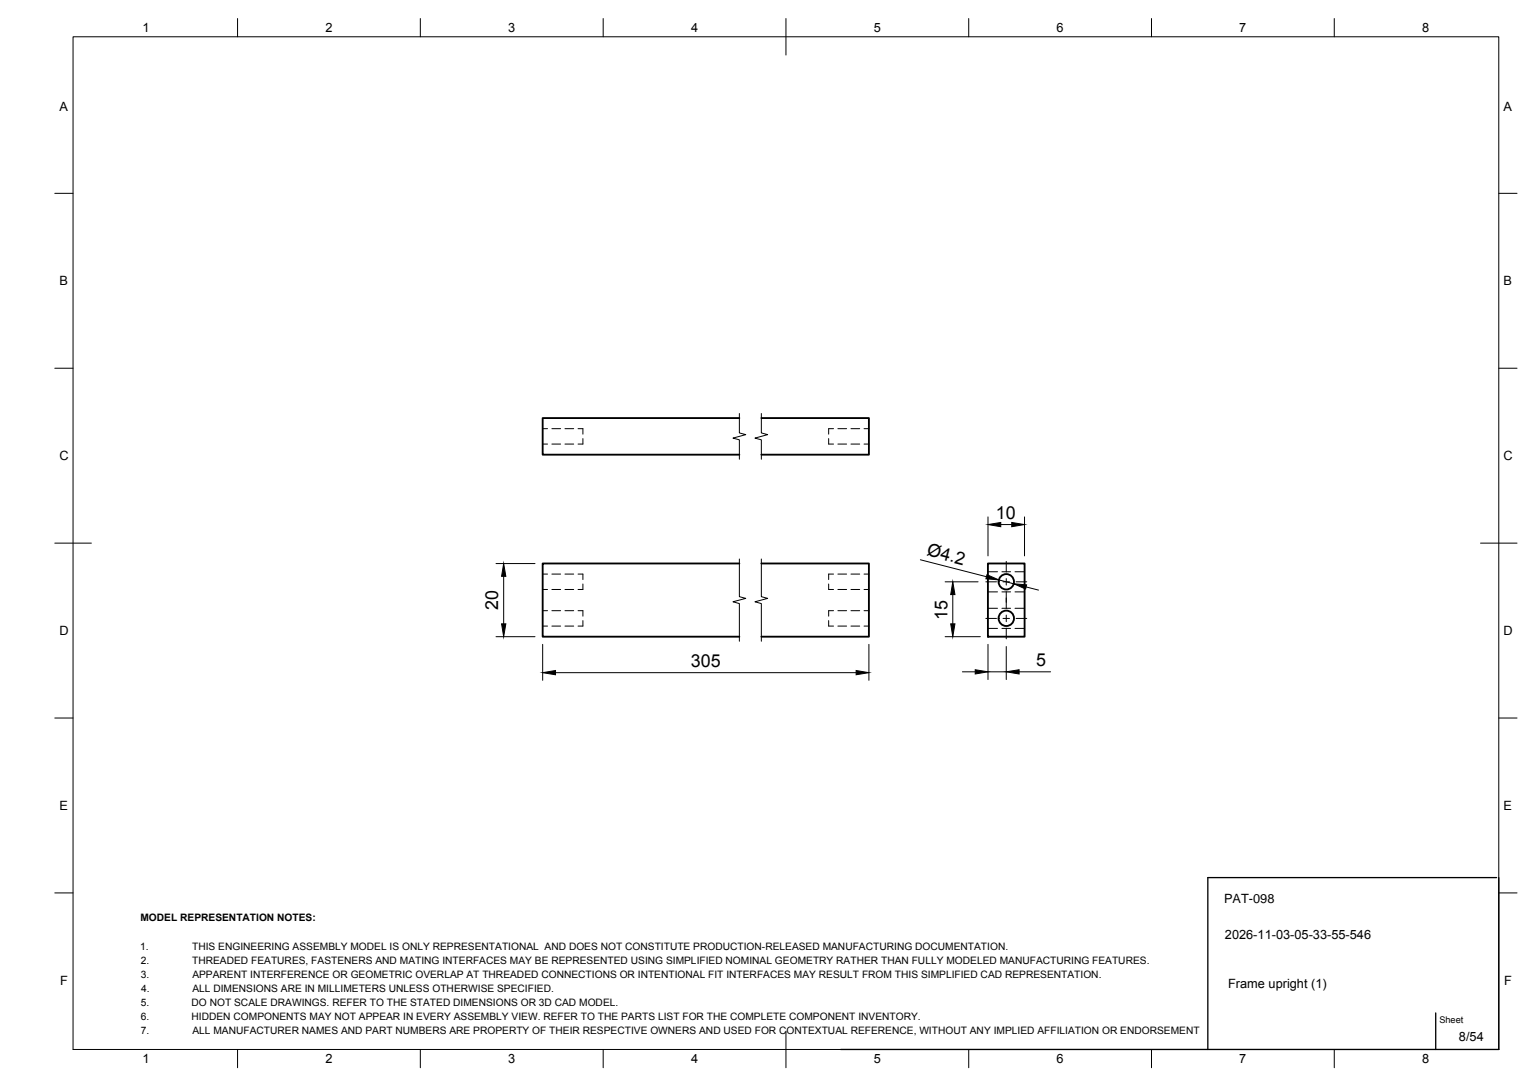
ISO-10303-21;
HEADER;
/* Generated by software containing ST-Developer
 * from STEP Tools, Inc. (www.steptools.com) 
 */

FILE_DESCRIPTION(
/* description */ ('Spring compression tester'),
/* implementation_level */ '2;1');

FILE_NAME(
/* name */ 'Frame upright (1).step',
/* time_stamp */ '2026-10-28T03:24:11-07:00',
/* author */ (''),
/* organization */ (''),
/* preprocessor_version */ 'ST-DEVELOPER v20.2',
/* originating_system */ 'Autodesk Translation Framework v15.17.0.0',
/* authorisation */ '');

FILE_SCHEMA (('AUTOMOTIVE_DESIGN { 1 0 10303 214 3 1 1 }'));
ENDSEC;

DATA;
#10=MECHANICAL_DESIGN_GEOMETRIC_PRESENTATION_REPRESENTATION('',(#1109),#43521);
#989=SHAPE_REPRESENTATION_RELATIONSHIP('SRR','None',#43801,#1049);
#1049=ADVANCED_BREP_SHAPE_REPRESENTATION('',(#1184),#43461);
#1109=STYLED_ITEM('',(#44181),#1184);
#1184=MANIFOLD_SOLID_BREP('Body1',#18546);
#1313=FACE_BOUND('',#3377,.T.);
#1314=FACE_BOUND('',#3378,.T.);
#1315=FACE_BOUND('',#3381,.T.);
#1316=FACE_BOUND('',#3382,.T.);
#1317=FACE_BOUND('',#3384,.T.);
#1318=FACE_BOUND('',#3385,.T.);
#1319=FACE_BOUND('',#3387,.T.);
#1320=FACE_BOUND('',#3388,.T.);
#1635=PLANE('',#19455);
#1636=PLANE('',#19459);
#1637=PLANE('',#19463);
#1638=PLANE('',#19467);
#1639=PLANE('',#19468);
#1640=PLANE('',#19469);
#1641=PLANE('',#19470);
#1642=PLANE('',#19471);
#1643=PLANE('',#19472);
#1644=PLANE('',#19473);
#2252=FACE_OUTER_BOUND('',#3365,.T.);
#2253=FACE_OUTER_BOUND('',#3366,.T.);
#2254=FACE_OUTER_BOUND('',#3367,.T.);
#2255=FACE_OUTER_BOUND('',#3368,.T.);
#2256=FACE_OUTER_BOUND('',#3369,.T.);
#2257=FACE_OUTER_BOUND('',#3370,.T.);
#2258=FACE_OUTER_BOUND('',#3371,.T.);
#2259=FACE_OUTER_BOUND('',#3372,.T.);
#2260=FACE_OUTER_BOUND('',#3373,.T.);
#2261=FACE_OUTER_BOUND('',#3374,.T.);
#2262=FACE_OUTER_BOUND('',#3375,.T.);
#2263=FACE_OUTER_BOUND('',#3376,.T.);
#2264=FACE_OUTER_BOUND('',#3379,.T.);
#2265=FACE_OUTER_BOUND('',#3380,.T.);
#2266=FACE_OUTER_BOUND('',#3383,.T.);
#2267=FACE_OUTER_BOUND('',#3386,.T.);
#3365=EDGE_LOOP('',(#12601,#12602,#12603,#12604));
#3366=EDGE_LOOP('',(#12605,#12606,#12607,#12608));
#3367=EDGE_LOOP('',(#12609,#12610,#12611,#12612));
#3368=EDGE_LOOP('',(#12613));
#3369=EDGE_LOOP('',(#12614,#12615,#12616,#12617));
#3370=EDGE_LOOP('',(#12618));
#3371=EDGE_LOOP('',(#12619,#12620,#12621,#12622));
#3372=EDGE_LOOP('',(#12623));
#3373=EDGE_LOOP('',(#12624,#12625,#12626,#12627));
#3374=EDGE_LOOP('',(#12628));
#3375=EDGE_LOOP('',(#12629,#12630,#12631,#12632));
#3376=EDGE_LOOP('',(#12633,#12634,#12635,#12636));
#3377=EDGE_LOOP('',(#12637));
#3378=EDGE_LOOP('',(#12638));
#3379=EDGE_LOOP('',(#12639,#12640,#12641,#12642));
#3380=EDGE_LOOP('',(#12643,#12644,#12645,#12646));
#3381=EDGE_LOOP('',(#12647));
#3382=EDGE_LOOP('',(#12648));
#3383=EDGE_LOOP('',(#12649,#12650,#12651,#12652));
#3384=EDGE_LOOP('',(#12653));
#3385=EDGE_LOOP('',(#12654));
#3386=EDGE_LOOP('',(#12655,#12656,#12657,#12658));
#3387=EDGE_LOOP('',(#12659));
#3388=EDGE_LOOP('',(#12660));
#4726=LINE('',#26866,#6158);
#4727=LINE('',#26872,#6159);
#4728=LINE('',#26878,#6160);
#4729=LINE('',#26885,#6161);
#4730=LINE('',#26892,#6162);
#4731=LINE('',#26899,#6163);
#4732=LINE('',#26905,#6164);
#4733=LINE('',#26907,#6165);
#4734=LINE('',#26909,#6166);
#4735=LINE('',#26910,#6167);
#4736=LINE('',#26913,#6168);
#4737=LINE('',#26915,#6169);
#4738=LINE('',#26916,#6170);
#4739=LINE('',#26919,#6171);
#4740=LINE('',#26921,#6172);
#4741=LINE('',#26922,#6173);
#4742=LINE('',#26924,#6174);
#4743=LINE('',#26925,#6175);
#6158=VECTOR('',#21644,0.274999999999999);
#6159=VECTOR('',#21651,0.274999999999999);
#6160=VECTOR('',#21658,0.21);
#6161=VECTOR('',#21667,0.21);
#6162=VECTOR('',#21676,0.21);
#6163=VECTOR('',#21685,0.21);
#6164=VECTOR('',#21692,1.);
#6165=VECTOR('',#21693,1.);
#6166=VECTOR('',#21694,1.);
#6167=VECTOR('',#21695,1.);
#6168=VECTOR('',#21698,1.);
#6169=VECTOR('',#21699,1.);
#6170=VECTOR('',#21700,1.);
#6171=VECTOR('',#21703,1.);
#6172=VECTOR('',#21704,1.);
#6173=VECTOR('',#21705,1.);
#6174=VECTOR('',#21708,1.);
#6175=VECTOR('',#21709,1.);
#7542=CIRCLE('',#19447,0.274999999999999);
#7543=CIRCLE('',#19448,0.274999999999999);
#7544=CIRCLE('',#19450,0.274999999999999);
#7545=CIRCLE('',#19451,0.274999999999999);
#7546=CIRCLE('',#19453,0.21);
#7547=CIRCLE('',#19454,0.21);
#7548=CIRCLE('',#19457,0.21);
#7549=CIRCLE('',#19458,0.21);
#7550=CIRCLE('',#19461,0.21);
#7551=CIRCLE('',#19462,0.21);
#7552=CIRCLE('',#19465,0.21);
#7553=CIRCLE('',#19466,0.21);
#8264=VERTEX_POINT('',#26863);
#8265=VERTEX_POINT('',#26865);
#8266=VERTEX_POINT('',#26869);
#8267=VERTEX_POINT('',#26871);
#8268=VERTEX_POINT('',#26875);
#8269=VERTEX_POINT('',#26877);
#8270=VERTEX_POINT('',#26882);
#8271=VERTEX_POINT('',#26884);
#8272=VERTEX_POINT('',#26889);
#8273=VERTEX_POINT('',#26891);
#8274=VERTEX_POINT('',#26896);
#8275=VERTEX_POINT('',#26898);
#8276=VERTEX_POINT('',#26903);
#8277=VERTEX_POINT('',#26904);
#8278=VERTEX_POINT('',#26906);
#8279=VERTEX_POINT('',#26908);
#8280=VERTEX_POINT('',#26912);
#8281=VERTEX_POINT('',#26914);
#8282=VERTEX_POINT('',#26918);
#8283=VERTEX_POINT('',#26920);
#9965=EDGE_CURVE('',#8264,#8264,#7542,.T.);
#9966=EDGE_CURVE('',#8264,#8265,#4726,.T.);
#9967=EDGE_CURVE('',#8265,#8265,#7543,.T.);
#9968=EDGE_CURVE('',#8266,#8266,#7544,.T.);
#9969=EDGE_CURVE('',#8266,#8267,#4727,.T.);
#9970=EDGE_CURVE('',#8267,#8267,#7545,.T.);
#9971=EDGE_CURVE('',#8268,#8268,#7546,.T.);
#9972=EDGE_CURVE('',#8268,#8269,#4728,.T.);
#9973=EDGE_CURVE('',#8269,#8269,#7547,.T.);
#9974=EDGE_CURVE('',#8270,#8270,#7548,.T.);
#9975=EDGE_CURVE('',#8270,#8271,#4729,.T.);
#9976=EDGE_CURVE('',#8271,#8271,#7549,.T.);
#9977=EDGE_CURVE('',#8272,#8272,#7550,.T.);
#9978=EDGE_CURVE('',#8272,#8273,#4730,.T.);
#9979=EDGE_CURVE('',#8273,#8273,#7551,.T.);
#9980=EDGE_CURVE('',#8274,#8274,#7552,.T.);
#9981=EDGE_CURVE('',#8274,#8275,#4731,.T.);
#9982=EDGE_CURVE('',#8275,#8275,#7553,.T.);
#9983=EDGE_CURVE('',#8276,#8277,#4732,.T.);
#9984=EDGE_CURVE('',#8277,#8278,#4733,.T.);
#9985=EDGE_CURVE('',#8279,#8278,#4734,.T.);
#9986=EDGE_CURVE('',#8276,#8279,#4735,.T.);
#9987=EDGE_CURVE('',#8280,#8276,#4736,.T.);
#9988=EDGE_CURVE('',#8281,#8279,#4737,.T.);
#9989=EDGE_CURVE('',#8280,#8281,#4738,.T.);
#9990=EDGE_CURVE('',#8282,#8280,#4739,.T.);
#9991=EDGE_CURVE('',#8283,#8281,#4740,.T.);
#9992=EDGE_CURVE('',#8282,#8283,#4741,.T.);
#9993=EDGE_CURVE('',#8277,#8282,#4742,.T.);
#9994=EDGE_CURVE('',#8278,#8283,#4743,.T.);
#12601=ORIENTED_EDGE('',*,*,#9965,.F.);
#12602=ORIENTED_EDGE('',*,*,#9966,.T.);
#12603=ORIENTED_EDGE('',*,*,#9967,.F.);
#12604=ORIENTED_EDGE('',*,*,#9966,.F.);
#12605=ORIENTED_EDGE('',*,*,#9968,.F.);
#12606=ORIENTED_EDGE('',*,*,#9969,.T.);
#12607=ORIENTED_EDGE('',*,*,#9970,.F.);
#12608=ORIENTED_EDGE('',*,*,#9969,.F.);
#12609=ORIENTED_EDGE('',*,*,#9971,.F.);
#12610=ORIENTED_EDGE('',*,*,#9972,.T.);
#12611=ORIENTED_EDGE('',*,*,#9973,.F.);
#12612=ORIENTED_EDGE('',*,*,#9972,.F.);
#12613=ORIENTED_EDGE('',*,*,#9971,.T.);
#12614=ORIENTED_EDGE('',*,*,#9974,.F.);
#12615=ORIENTED_EDGE('',*,*,#9975,.T.);
#12616=ORIENTED_EDGE('',*,*,#9976,.F.);
#12617=ORIENTED_EDGE('',*,*,#9975,.F.);
#12618=ORIENTED_EDGE('',*,*,#9974,.T.);
#12619=ORIENTED_EDGE('',*,*,#9977,.F.);
#12620=ORIENTED_EDGE('',*,*,#9978,.T.);
#12621=ORIENTED_EDGE('',*,*,#9979,.T.);
#12622=ORIENTED_EDGE('',*,*,#9978,.F.);
#12623=ORIENTED_EDGE('',*,*,#9979,.F.);
#12624=ORIENTED_EDGE('',*,*,#9980,.F.);
#12625=ORIENTED_EDGE('',*,*,#9981,.T.);
#12626=ORIENTED_EDGE('',*,*,#9982,.T.);
#12627=ORIENTED_EDGE('',*,*,#9981,.F.);
#12628=ORIENTED_EDGE('',*,*,#9982,.F.);
#12629=ORIENTED_EDGE('',*,*,#9983,.T.);
#12630=ORIENTED_EDGE('',*,*,#9984,.T.);
#12631=ORIENTED_EDGE('',*,*,#9985,.F.);
#12632=ORIENTED_EDGE('',*,*,#9986,.F.);
#12633=ORIENTED_EDGE('',*,*,#9987,.T.);
#12634=ORIENTED_EDGE('',*,*,#9986,.T.);
#12635=ORIENTED_EDGE('',*,*,#9988,.F.);
#12636=ORIENTED_EDGE('',*,*,#9989,.F.);
#12637=ORIENTED_EDGE('',*,*,#9967,.T.);
#12638=ORIENTED_EDGE('',*,*,#9970,.T.);
#12639=ORIENTED_EDGE('',*,*,#9990,.T.);
#12640=ORIENTED_EDGE('',*,*,#9989,.T.);
#12641=ORIENTED_EDGE('',*,*,#9991,.F.);
#12642=ORIENTED_EDGE('',*,*,#9992,.F.);
#12643=ORIENTED_EDGE('',*,*,#9993,.T.);
#12644=ORIENTED_EDGE('',*,*,#9992,.T.);
#12645=ORIENTED_EDGE('',*,*,#9994,.F.);
#12646=ORIENTED_EDGE('',*,*,#9984,.F.);
#12647=ORIENTED_EDGE('',*,*,#9965,.T.);
#12648=ORIENTED_EDGE('',*,*,#9968,.T.);
#12649=ORIENTED_EDGE('',*,*,#9994,.T.);
#12650=ORIENTED_EDGE('',*,*,#9991,.T.);
#12651=ORIENTED_EDGE('',*,*,#9988,.T.);
#12652=ORIENTED_EDGE('',*,*,#9985,.T.);
#12653=ORIENTED_EDGE('',*,*,#9973,.T.);
#12654=ORIENTED_EDGE('',*,*,#9976,.T.);
#12655=ORIENTED_EDGE('',*,*,#9993,.F.);
#12656=ORIENTED_EDGE('',*,*,#9983,.F.);
#12657=ORIENTED_EDGE('',*,*,#9987,.F.);
#12658=ORIENTED_EDGE('',*,*,#9990,.F.);
#12659=ORIENTED_EDGE('',*,*,#9977,.T.);
#12660=ORIENTED_EDGE('',*,*,#9980,.T.);
#17141=CYLINDRICAL_SURFACE('',#19446,0.274999999999999);
#17142=CYLINDRICAL_SURFACE('',#19449,0.274999999999999);
#17143=CYLINDRICAL_SURFACE('',#19452,0.21);
#17144=CYLINDRICAL_SURFACE('',#19456,0.21);
#17145=CYLINDRICAL_SURFACE('',#19460,0.21);
#17146=CYLINDRICAL_SURFACE('',#19464,0.21);
#17576=ADVANCED_FACE('',(#2252),#17141,.F.);
#17577=ADVANCED_FACE('',(#2253),#17142,.F.);
#17578=ADVANCED_FACE('',(#2254),#17143,.F.);
#17579=ADVANCED_FACE('',(#2255),#1635,.T.);
#17580=ADVANCED_FACE('',(#2256),#17144,.F.);
#17581=ADVANCED_FACE('',(#2257),#1636,.T.);
#17582=ADVANCED_FACE('',(#2258),#17145,.F.);
#17583=ADVANCED_FACE('',(#2259),#1637,.F.);
#17584=ADVANCED_FACE('',(#2260),#17146,.F.);
#17585=ADVANCED_FACE('',(#2261),#1638,.F.);
#17586=ADVANCED_FACE('',(#2262),#1639,.T.);
#17587=ADVANCED_FACE('',(#2263,#1313,#1314),#1640,.T.);
#17588=ADVANCED_FACE('',(#2264),#1641,.T.);
#17589=ADVANCED_FACE('',(#2265,#1315,#1316),#1642,.T.);
#17590=ADVANCED_FACE('',(#2266,#1317,#1318),#1643,.T.);
#17591=ADVANCED_FACE('',(#2267,#1319,#1320),#1644,.F.);
#18546=CLOSED_SHELL('',(#17576,#17577,#17578,#17579,#17580,#17581,#17582,
#17583,#17584,#17585,#17586,#17587,#17588,#17589,#17590,#17591));
#19445=AXIS2_PLACEMENT_3D('',#26861,#21638,#21639);
#19446=AXIS2_PLACEMENT_3D('',#26862,#21640,#21641);
#19447=AXIS2_PLACEMENT_3D('',#26864,#21642,#21643);
#19448=AXIS2_PLACEMENT_3D('',#26867,#21645,#21646);
#19449=AXIS2_PLACEMENT_3D('',#26868,#21647,#21648);
#19450=AXIS2_PLACEMENT_3D('',#26870,#21649,#21650);
#19451=AXIS2_PLACEMENT_3D('',#26873,#21652,#21653);
#19452=AXIS2_PLACEMENT_3D('',#26874,#21654,#21655);
#19453=AXIS2_PLACEMENT_3D('',#26876,#21656,#21657);
#19454=AXIS2_PLACEMENT_3D('',#26879,#21659,#21660);
#19455=AXIS2_PLACEMENT_3D('',#26880,#21661,#21662);
#19456=AXIS2_PLACEMENT_3D('',#26881,#21663,#21664);
#19457=AXIS2_PLACEMENT_3D('',#26883,#21665,#21666);
#19458=AXIS2_PLACEMENT_3D('',#26886,#21668,#21669);
#19459=AXIS2_PLACEMENT_3D('',#26887,#21670,#21671);
#19460=AXIS2_PLACEMENT_3D('',#26888,#21672,#21673);
#19461=AXIS2_PLACEMENT_3D('',#26890,#21674,#21675);
#19462=AXIS2_PLACEMENT_3D('',#26893,#21677,#21678);
#19463=AXIS2_PLACEMENT_3D('',#26894,#21679,#21680);
#19464=AXIS2_PLACEMENT_3D('',#26895,#21681,#21682);
#19465=AXIS2_PLACEMENT_3D('',#26897,#21683,#21684);
#19466=AXIS2_PLACEMENT_3D('',#26900,#21686,#21687);
#19467=AXIS2_PLACEMENT_3D('',#26901,#21688,#21689);
#19468=AXIS2_PLACEMENT_3D('',#26902,#21690,#21691);
#19469=AXIS2_PLACEMENT_3D('',#26911,#21696,#21697);
#19470=AXIS2_PLACEMENT_3D('',#26917,#21701,#21702);
#19471=AXIS2_PLACEMENT_3D('',#26923,#21706,#21707);
#19472=AXIS2_PLACEMENT_3D('',#26926,#21710,#21711);
#19473=AXIS2_PLACEMENT_3D('',#26927,#21712,#21713);
#21638=DIRECTION('axis',(0.,0.,1.));
#21639=DIRECTION('refdir',(1.,0.,0.));
#21640=DIRECTION('center_axis',(1.,0.,0.));
#21641=DIRECTION('ref_axis',(0.,0.,-1.));
#21642=DIRECTION('center_axis',(1.,0.,0.));
#21643=DIRECTION('ref_axis',(0.,0.,-1.));
#21644=DIRECTION('',(1.,0.,0.));
#21645=DIRECTION('center_axis',(-1.,0.,0.));
#21646=DIRECTION('ref_axis',(0.,0.,-1.));
#21647=DIRECTION('center_axis',(1.,0.,0.));
#21648=DIRECTION('ref_axis',(0.,0.,-1.));
#21649=DIRECTION('center_axis',(1.,0.,0.));
#21650=DIRECTION('ref_axis',(0.,0.,-1.));
#21651=DIRECTION('',(1.,0.,0.));
#21652=DIRECTION('center_axis',(-1.,0.,0.));
#21653=DIRECTION('ref_axis',(0.,0.,-1.));
#21654=DIRECTION('center_axis',(0.,0.,1.));
#21655=DIRECTION('ref_axis',(1.,0.,0.));
#21656=DIRECTION('center_axis',(0.,0.,1.));
#21657=DIRECTION('ref_axis',(1.,0.,0.));
#21658=DIRECTION('',(0.,0.,1.));
#21659=DIRECTION('center_axis',(0.,0.,-1.));
#21660=DIRECTION('ref_axis',(1.,0.,0.));
#21661=DIRECTION('center_axis',(0.,0.,1.));
#21662=DIRECTION('ref_axis',(1.,0.,0.));
#21663=DIRECTION('center_axis',(0.,0.,1.));
#21664=DIRECTION('ref_axis',(1.,0.,0.));
#21665=DIRECTION('center_axis',(0.,0.,1.));
#21666=DIRECTION('ref_axis',(1.,0.,0.));
#21667=DIRECTION('',(0.,0.,1.));
#21668=DIRECTION('center_axis',(0.,0.,-1.));
#21669=DIRECTION('ref_axis',(1.,0.,0.));
#21670=DIRECTION('center_axis',(0.,0.,1.));
#21671=DIRECTION('ref_axis',(1.,0.,0.));
#21672=DIRECTION('center_axis',(0.,0.,1.));
#21673=DIRECTION('ref_axis',(1.,0.,0.));
#21674=DIRECTION('center_axis',(0.,0.,1.));
#21675=DIRECTION('ref_axis',(1.,0.,0.));
#21676=DIRECTION('',(0.,0.,1.));
#21677=DIRECTION('center_axis',(0.,0.,1.));
#21678=DIRECTION('ref_axis',(1.,0.,0.));
#21679=DIRECTION('center_axis',(0.,0.,1.));
#21680=DIRECTION('ref_axis',(1.,0.,0.));
#21681=DIRECTION('center_axis',(0.,0.,1.));
#21682=DIRECTION('ref_axis',(1.,0.,0.));
#21683=DIRECTION('center_axis',(0.,0.,1.));
#21684=DIRECTION('ref_axis',(1.,0.,0.));
#21685=DIRECTION('',(0.,0.,1.));
#21686=DIRECTION('center_axis',(0.,0.,1.));
#21687=DIRECTION('ref_axis',(1.,0.,0.));
#21688=DIRECTION('center_axis',(0.,0.,1.));
#21689=DIRECTION('ref_axis',(1.,0.,0.));
#21690=DIRECTION('center_axis',(0.,1.,0.));
#21691=DIRECTION('ref_axis',(-1.,0.,0.));
#21692=DIRECTION('',(-1.,0.,0.));
#21693=DIRECTION('',(0.,0.,1.));
#21694=DIRECTION('',(-1.,0.,0.));
#21695=DIRECTION('',(0.,0.,1.));
#21696=DIRECTION('center_axis',(1.,0.,0.));
#21697=DIRECTION('ref_axis',(0.,1.,0.));
#21698=DIRECTION('',(0.,1.,0.));
#21699=DIRECTION('',(0.,1.,0.));
#21700=DIRECTION('',(0.,0.,1.));
#21701=DIRECTION('center_axis',(0.,-1.,0.));
#21702=DIRECTION('ref_axis',(1.,0.,0.));
#21703=DIRECTION('',(1.,0.,0.));
#21704=DIRECTION('',(1.,0.,0.));
#21705=DIRECTION('',(0.,0.,1.));
#21706=DIRECTION('center_axis',(-1.,0.,0.));
#21707=DIRECTION('ref_axis',(0.,-1.,0.));
#21708=DIRECTION('',(0.,-1.,0.));
#21709=DIRECTION('',(0.,-1.,0.));
#21710=DIRECTION('center_axis',(0.,0.,1.));
#21711=DIRECTION('ref_axis',(1.,0.,0.));
#21712=DIRECTION('center_axis',(0.,0.,1.));
#21713=DIRECTION('ref_axis',(1.,0.,0.));
#26861=CARTESIAN_POINT('',(0.,0.,0.));
#26862=CARTESIAN_POINT('Origin',(6.4,9.5,24.));
#26863=CARTESIAN_POINT('',(6.5,9.5,24.275));
#26864=CARTESIAN_POINT('Origin',(6.5,9.5,24.));
#26865=CARTESIAN_POINT('',(7.5,9.5,24.275));
#26866=CARTESIAN_POINT('',(6.4,9.5,24.275));
#26867=CARTESIAN_POINT('Origin',(7.5,9.5,24.));
#26868=CARTESIAN_POINT('Origin',(6.4,10.5,24.));
#26869=CARTESIAN_POINT('',(6.5,10.5,24.275));
#26870=CARTESIAN_POINT('Origin',(6.5,10.5,24.));
#26871=CARTESIAN_POINT('',(7.5,10.5,24.275));
#26872=CARTESIAN_POINT('',(6.4,10.5,24.275));
#26873=CARTESIAN_POINT('Origin',(7.5,10.5,24.));
#26874=CARTESIAN_POINT('Origin',(7.,9.5,29.4));
#26875=CARTESIAN_POINT('',(6.79,9.5,29.4));
#26876=CARTESIAN_POINT('Origin',(7.,9.5,29.4));
#26877=CARTESIAN_POINT('',(6.79,9.5,30.5));
#26878=CARTESIAN_POINT('',(6.79,9.5,29.4));
#26879=CARTESIAN_POINT('Origin',(7.,9.5,30.5));
#26880=CARTESIAN_POINT('Origin',(7.,9.5,29.4));
#26881=CARTESIAN_POINT('Origin',(7.,10.5,29.4));
#26882=CARTESIAN_POINT('',(6.79,10.5,29.4));
#26883=CARTESIAN_POINT('Origin',(7.,10.5,29.4));
#26884=CARTESIAN_POINT('',(6.79,10.5,30.5));
#26885=CARTESIAN_POINT('',(6.79,10.5,29.4));
#26886=CARTESIAN_POINT('Origin',(7.,10.5,30.5));
#26887=CARTESIAN_POINT('Origin',(7.,10.5,29.4));
#26888=CARTESIAN_POINT('Origin',(7.,9.5,-0.1));
#26889=CARTESIAN_POINT('',(6.79,9.5,0.));
#26890=CARTESIAN_POINT('Origin',(7.,9.5,0.));
#26891=CARTESIAN_POINT('',(6.79,9.5,1.1));
#26892=CARTESIAN_POINT('',(6.79,9.5,-0.1));
#26893=CARTESIAN_POINT('Origin',(7.,9.5,1.1));
#26894=CARTESIAN_POINT('Origin',(7.,9.5,1.1));
#26895=CARTESIAN_POINT('Origin',(7.,10.5,-0.1));
#26896=CARTESIAN_POINT('',(6.79,10.5,0.));
#26897=CARTESIAN_POINT('Origin',(7.,10.5,0.));
#26898=CARTESIAN_POINT('',(6.79,10.5,1.1));
#26899=CARTESIAN_POINT('',(6.79,10.5,-0.1));
#26900=CARTESIAN_POINT('Origin',(7.,10.5,1.1));
#26901=CARTESIAN_POINT('Origin',(7.,10.5,1.1));
#26902=CARTESIAN_POINT('Origin',(7.5,11.,0.));
#26903=CARTESIAN_POINT('',(7.5,11.,0.));
#26904=CARTESIAN_POINT('',(6.5,11.,0.));
#26905=CARTESIAN_POINT('',(7.5,11.,0.));
#26906=CARTESIAN_POINT('',(6.5,11.,30.5));
#26907=CARTESIAN_POINT('',(6.5,11.,0.));
#26908=CARTESIAN_POINT('',(7.5,11.,30.5));
#26909=CARTESIAN_POINT('',(7.5,11.,30.5));
#26910=CARTESIAN_POINT('',(7.5,11.,0.));
#26911=CARTESIAN_POINT('Origin',(7.5,9.,0.));
#26912=CARTESIAN_POINT('',(7.5,9.,0.));
#26913=CARTESIAN_POINT('',(7.5,9.,0.));
#26914=CARTESIAN_POINT('',(7.5,9.,30.5));
#26915=CARTESIAN_POINT('',(7.5,9.,30.5));
#26916=CARTESIAN_POINT('',(7.5,9.,0.));
#26917=CARTESIAN_POINT('Origin',(6.5,9.,0.));
#26918=CARTESIAN_POINT('',(6.5,9.,0.));
#26919=CARTESIAN_POINT('',(6.5,9.,0.));
#26920=CARTESIAN_POINT('',(6.5,9.,30.5));
#26921=CARTESIAN_POINT('',(6.5,9.,30.5));
#26922=CARTESIAN_POINT('',(6.5,9.,0.));
#26923=CARTESIAN_POINT('Origin',(6.5,11.,0.));
#26924=CARTESIAN_POINT('',(6.5,11.,0.));
#26925=CARTESIAN_POINT('',(6.5,11.,30.5));
#26926=CARTESIAN_POINT('Origin',(7.,10.,30.5));
#26927=CARTESIAN_POINT('Origin',(7.,10.,0.));
#43393=UNCERTAINTY_MEASURE_WITH_UNIT(LENGTH_MEASURE(0.001),#43522,
'DISTANCE_ACCURACY_VALUE',
'Maximum model space distance between geometric entities at asserted c
onnectivities');
#43453=UNCERTAINTY_MEASURE_WITH_UNIT(LENGTH_MEASURE(0.001),#43522,
'DISTANCE_ACCURACY_VALUE',
'Maximum model space distance between geometric entities at asserted c
onnectivities');
#43461=(
GEOMETRIC_REPRESENTATION_CONTEXT(3)
GLOBAL_UNCERTAINTY_ASSIGNED_CONTEXT((#43393))
GLOBAL_UNIT_ASSIGNED_CONTEXT((#43522,#43524,#43525))
REPRESENTATION_CONTEXT('','3D')
);
#43521=(
GEOMETRIC_REPRESENTATION_CONTEXT(3)
GLOBAL_UNCERTAINTY_ASSIGNED_CONTEXT((#43453))
GLOBAL_UNIT_ASSIGNED_CONTEXT((#43522,#43524,#43525))
REPRESENTATION_CONTEXT('','3D')
);
#43522=(
LENGTH_UNIT()
NAMED_UNIT(*)
SI_UNIT(.CENTI.,.METRE.)
);
#43524=(
NAMED_UNIT(*)
PLANE_ANGLE_UNIT()
SI_UNIT($,.RADIAN.)
);
#43525=(
NAMED_UNIT(*)
SI_UNIT($,.STERADIAN.)
SOLID_ANGLE_UNIT()
);
#43533=SHAPE_DEFINITION_REPRESENTATION(#43600,#43801);
#43600=PRODUCT_DEFINITION_SHAPE('',$,#43869);
#43801=SHAPE_REPRESENTATION('',(#19445),#43461);
#43861=PRODUCT_DEFINITION_CONTEXT('part definition',#44064,'design');
#43869=PRODUCT_DEFINITION('Frame upright (1)','Frame upright (1)',#43936,
#43861);
#43936=PRODUCT_DEFINITION_FORMATION('',$,#44073);
#44064=APPLICATION_CONTEXT(
'Core Data for Automotive Mechanical Design Process');
#44065=PRODUCT_CONTEXT('part definition',#44064,'mechanical');
#44073=PRODUCT('Frame upright (1)','Frame upright (1)','Frame upright (1)',(#44065));
#44175=COLOUR_RGB('Dark Blue',0.08,0.2,0.34);
#44176=FILL_AREA_STYLE_COLOUR('',#44175);
#44177=FILL_AREA_STYLE('',(#44176));
#44178=SURFACE_STYLE_FILL_AREA(#44177);
#44179=SURFACE_SIDE_STYLE('',(#44178));
#44180=SURFACE_STYLE_USAGE(.BOTH.,#44179);
#44181=PRESENTATION_STYLE_ASSIGNMENT((#44180));
ENDSEC;
END-ISO-10303-21;
